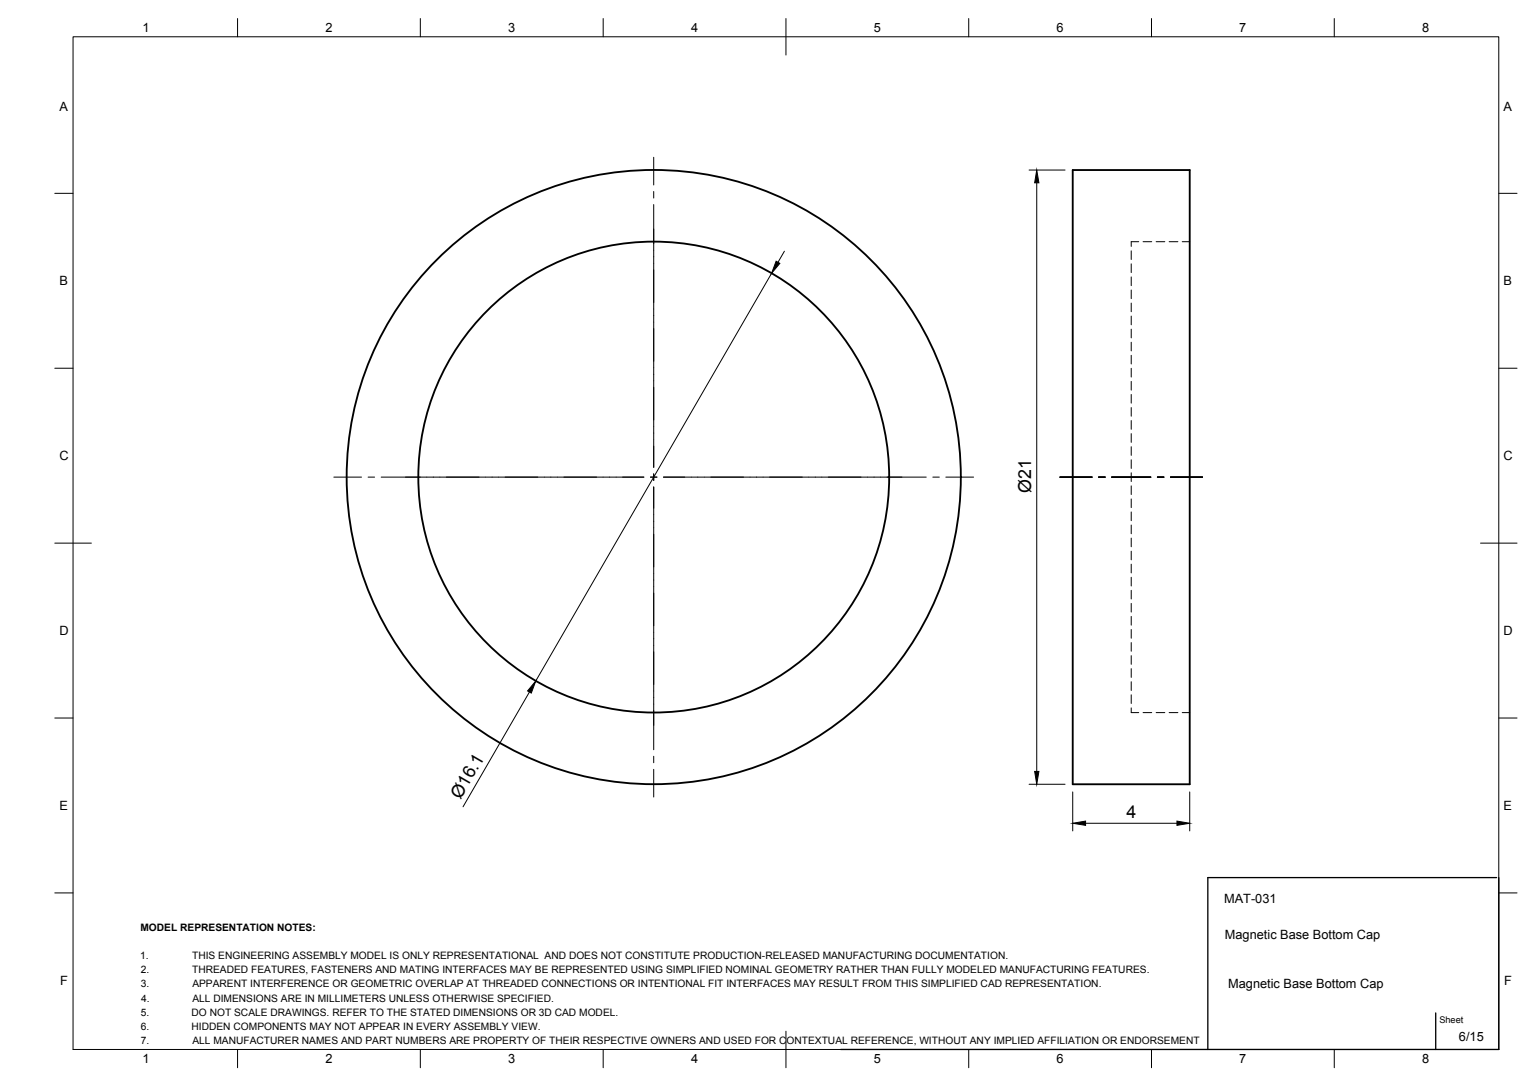
ISO-10303-21;
HEADER;
/* Generated by software containing ST-Developer
 * from STEP Tools, Inc. (www.steptools.com) 
 */

FILE_DESCRIPTION(
/* description */ ('STEP AP214'),
/* implementation_level */ '2;1');

FILE_NAME(
/* name */ 'Magnetic Base Bottom Cap.step',
/* time_stamp */ '2026-11-14T06:58:01-08:00',
/* author */ (''),
/* organization */ (''),
/* preprocessor_version */ 'ST-DEVELOPER v20.2',
/* originating_system */ 'Autodesk Translation Framework v15.17.0.0',
/* authorisation */ '');

FILE_SCHEMA (('AUTOMOTIVE_DESIGN { 1 0 10303 214 3 1 1 }'));
ENDSEC;

DATA;
#10=MECHANICAL_DESIGN_GEOMETRIC_PRESENTATION_REPRESENTATION('',(#1149),#38635);
#869=FACE_BOUND('',#2800,.T.);
#1115=SHAPE_REPRESENTATION_RELATIONSHIP('SRR','None',#38688,#1129);
#1129=ADVANCED_BREP_SHAPE_REPRESENTATION('',(#1175),#38624);
#1149=STYLED_ITEM('',(#38766),#1175);
#1175=MANIFOLD_SOLID_BREP('Body1',#17615);
#1245=PLANE('',#18009);
#1246=PLANE('',#18010);
#1247=PLANE('',#18011);
#1783=FACE_OUTER_BOUND('',#2796,.T.);
#1784=FACE_OUTER_BOUND('',#2797,.T.);
#1785=FACE_OUTER_BOUND('',#2798,.T.);
#1786=FACE_OUTER_BOUND('',#2799,.T.);
#1787=FACE_OUTER_BOUND('',#2801,.T.);
#2796=EDGE_LOOP('',(#11625,#11626,#11627,#11628));
#2797=EDGE_LOOP('',(#11629,#11630,#11631,#11632));
#2798=EDGE_LOOP('',(#11633));
#2799=EDGE_LOOP('',(#11634));
#2800=EDGE_LOOP('',(#11635));
#2801=EDGE_LOOP('',(#11636));
#3873=LINE('',#29891,#4817);
#3874=LINE('',#29897,#4818);
#4817=VECTOR('',#20354,8.05);
#4818=VECTOR('',#20361,10.5);
#5659=CIRCLE('',#18004,8.05);
#5660=CIRCLE('',#18005,8.05);
#5661=CIRCLE('',#18007,10.5);
#5662=CIRCLE('',#18008,10.5);
#6749=VERTEX_POINT('',#29888);
#6750=VERTEX_POINT('',#29890);
#6751=VERTEX_POINT('',#29894);
#6752=VERTEX_POINT('',#29896);
#8599=EDGE_CURVE('',#6749,#6749,#5659,.T.);
#8600=EDGE_CURVE('',#6749,#6750,#3873,.T.);
#8601=EDGE_CURVE('',#6750,#6750,#5660,.T.);
#8602=EDGE_CURVE('',#6751,#6751,#5661,.T.);
#8603=EDGE_CURVE('',#6751,#6752,#3874,.T.);
#8604=EDGE_CURVE('',#6752,#6752,#5662,.T.);
#11625=ORIENTED_EDGE('',*,*,#8599,.T.);
#11626=ORIENTED_EDGE('',*,*,#8600,.T.);
#11627=ORIENTED_EDGE('',*,*,#8601,.T.);
#11628=ORIENTED_EDGE('',*,*,#8600,.F.);
#11629=ORIENTED_EDGE('',*,*,#8602,.T.);
#11630=ORIENTED_EDGE('',*,*,#8603,.T.);
#11631=ORIENTED_EDGE('',*,*,#8604,.F.);
#11632=ORIENTED_EDGE('',*,*,#8603,.F.);
#11633=ORIENTED_EDGE('',*,*,#8602,.F.);
#11634=ORIENTED_EDGE('',*,*,#8604,.T.);
#11635=ORIENTED_EDGE('',*,*,#8599,.F.);
#11636=ORIENTED_EDGE('',*,*,#8601,.F.);
#16323=CYLINDRICAL_SURFACE('',#18003,8.05);
#16324=CYLINDRICAL_SURFACE('',#18006,10.5);
#16742=ADVANCED_FACE('',(#1783),#16323,.F.);
#16743=ADVANCED_FACE('',(#1784),#16324,.T.);
#16744=ADVANCED_FACE('',(#1785),#1245,.F.);
#16745=ADVANCED_FACE('',(#1786,#869),#1246,.T.);
#16746=ADVANCED_FACE('',(#1787),#1247,.T.);
#17615=CLOSED_SHELL('',(#16742,#16743,#16744,#16745,#16746));
#18002=AXIS2_PLACEMENT_3D('',#29886,#20348,#20349);
#18003=AXIS2_PLACEMENT_3D('',#29887,#20350,#20351);
#18004=AXIS2_PLACEMENT_3D('',#29889,#20352,#20353);
#18005=AXIS2_PLACEMENT_3D('',#29892,#20355,#20356);
#18006=AXIS2_PLACEMENT_3D('',#29893,#20357,#20358);
#18007=AXIS2_PLACEMENT_3D('',#29895,#20359,#20360);
#18008=AXIS2_PLACEMENT_3D('',#29898,#20362,#20363);
#18009=AXIS2_PLACEMENT_3D('',#29899,#20364,#20365);
#18010=AXIS2_PLACEMENT_3D('',#29900,#20366,#20367);
#18011=AXIS2_PLACEMENT_3D('',#29901,#20368,#20369);
#20348=DIRECTION('axis',(0.,0.,1.));
#20349=DIRECTION('refdir',(1.,0.,0.));
#20350=DIRECTION('center_axis',(0.,-1.,0.));
#20351=DIRECTION('ref_axis',(0.,0.,-1.));
#20352=DIRECTION('center_axis',(0.,1.,0.));
#20353=DIRECTION('ref_axis',(0.,0.,1.));
#20354=DIRECTION('',(0.,-1.,0.));
#20355=DIRECTION('center_axis',(0.,-1.,0.));
#20356=DIRECTION('ref_axis',(0.,0.,1.));
#20357=DIRECTION('center_axis',(0.,-1.,0.));
#20358=DIRECTION('ref_axis',(0.,0.,-1.));
#20359=DIRECTION('center_axis',(0.,1.,0.));
#20360=DIRECTION('ref_axis',(0.,0.,1.));
#20361=DIRECTION('',(0.,1.,0.));
#20362=DIRECTION('center_axis',(0.,1.,0.));
#20363=DIRECTION('ref_axis',(0.,0.,1.));
#20364=DIRECTION('center_axis',(0.,1.,0.));
#20365=DIRECTION('ref_axis',(0.,0.,1.));
#20366=DIRECTION('center_axis',(0.,1.,0.));
#20367=DIRECTION('ref_axis',(0.,0.,1.));
#20368=DIRECTION('center_axis',(0.,1.,0.));
#20369=DIRECTION('ref_axis',(0.,0.,1.));
#29886=CARTESIAN_POINT('',(0.,0.,0.));
#29887=CARTESIAN_POINT('Origin',(0.,4.,0.));
#29888=CARTESIAN_POINT('',(-9.85840673313619E-16,4.,8.05));
#29889=CARTESIAN_POINT('Origin',(0.,4.,0.));
#29890=CARTESIAN_POINT('',(-9.85840673313619E-16,2.,8.05));
#29891=CARTESIAN_POINT('',(-9.85840673313619E-16,4.,8.05));
#29892=CARTESIAN_POINT('Origin',(0.,2.,0.));
#29893=CARTESIAN_POINT('Origin',(0.,2.,0.));
#29894=CARTESIAN_POINT('',(-1.28587913910472E-15,0.,10.5));
#29895=CARTESIAN_POINT('Origin',(0.,0.,0.));
#29896=CARTESIAN_POINT('',(-1.28587913910472E-15,4.,10.5));
#29897=CARTESIAN_POINT('',(-1.28587913910472E-15,2.,10.5));
#29898=CARTESIAN_POINT('Origin',(0.,4.,0.));
#29899=CARTESIAN_POINT('Origin',(0.,0.,0.));
#29900=CARTESIAN_POINT('Origin',(0.,4.,0.));
#29901=CARTESIAN_POINT('Origin',(0.,2.,0.));
#38608=UNCERTAINTY_MEASURE_WITH_UNIT(LENGTH_MEASURE(0.01),#38636,
'DISTANCE_ACCURACY_VALUE',
'Maximum model space distance between geometric entities at asserted c
onnectivities');
#38619=UNCERTAINTY_MEASURE_WITH_UNIT(LENGTH_MEASURE(0.01),#38636,
'DISTANCE_ACCURACY_VALUE',
'Maximum model space distance between geometric entities at asserted c
onnectivities');
#38624=(
GEOMETRIC_REPRESENTATION_CONTEXT(3)
GLOBAL_UNCERTAINTY_ASSIGNED_CONTEXT((#38608))
GLOBAL_UNIT_ASSIGNED_CONTEXT((#38636,#38638,#38639))
REPRESENTATION_CONTEXT('','3D')
);
#38635=(
GEOMETRIC_REPRESENTATION_CONTEXT(3)
GLOBAL_UNCERTAINTY_ASSIGNED_CONTEXT((#38619))
GLOBAL_UNIT_ASSIGNED_CONTEXT((#38636,#38638,#38639))
REPRESENTATION_CONTEXT('','3D')
);
#38636=(
LENGTH_UNIT()
NAMED_UNIT(*)
SI_UNIT(.MILLI.,.METRE.)
);
#38638=(
NAMED_UNIT(*)
PLANE_ANGLE_UNIT()
SI_UNIT($,.RADIAN.)
);
#38639=(
NAMED_UNIT(*)
SI_UNIT($,.STERADIAN.)
SOLID_ANGLE_UNIT()
);
#38644=SHAPE_DEFINITION_REPRESENTATION(#38659,#38688);
#38659=PRODUCT_DEFINITION_SHAPE('',$,#38704);
#38688=SHAPE_REPRESENTATION('',(#18002),#38624);
#38699=PRODUCT_DEFINITION_CONTEXT('part definition',#38746,'design');
#38704=PRODUCT_DEFINITION('Magnetic Base Bottom Cap',
'Magnetic Base Bottom Cap',#38719,#38699);
#38719=PRODUCT_DEFINITION_FORMATION('',$,#38752);
#38746=APPLICATION_CONTEXT(
'Core Data for Automotive Mechanical Design Process');
#38747=PRODUCT_CONTEXT('part definition',#38746,'mechanical');
#38752=PRODUCT('Magnetic Base Bottom Cap','Magnetic Base Bottom Cap',$,
(#38747));
#38766=PRESENTATION_STYLE_ASSIGNMENT((#38773));
#38773=SURFACE_STYLE_USAGE(.BOTH.,#38780);
#38780=SURFACE_SIDE_STYLE('',(#38787));
#38787=SURFACE_STYLE_FILL_AREA(#38794);
#38794=FILL_AREA_STYLE('Opaque(61,176,222)',(#38801));
#38801=FILL_AREA_STYLE_COLOUR('Opaque(61,176,222)',#38808);
#38808=COLOUR_RGB('Opaque(61,176,222)',0.23921568627451,0.690196078431373,
0.870588235294118);
ENDSEC;
END-ISO-10303-21;
